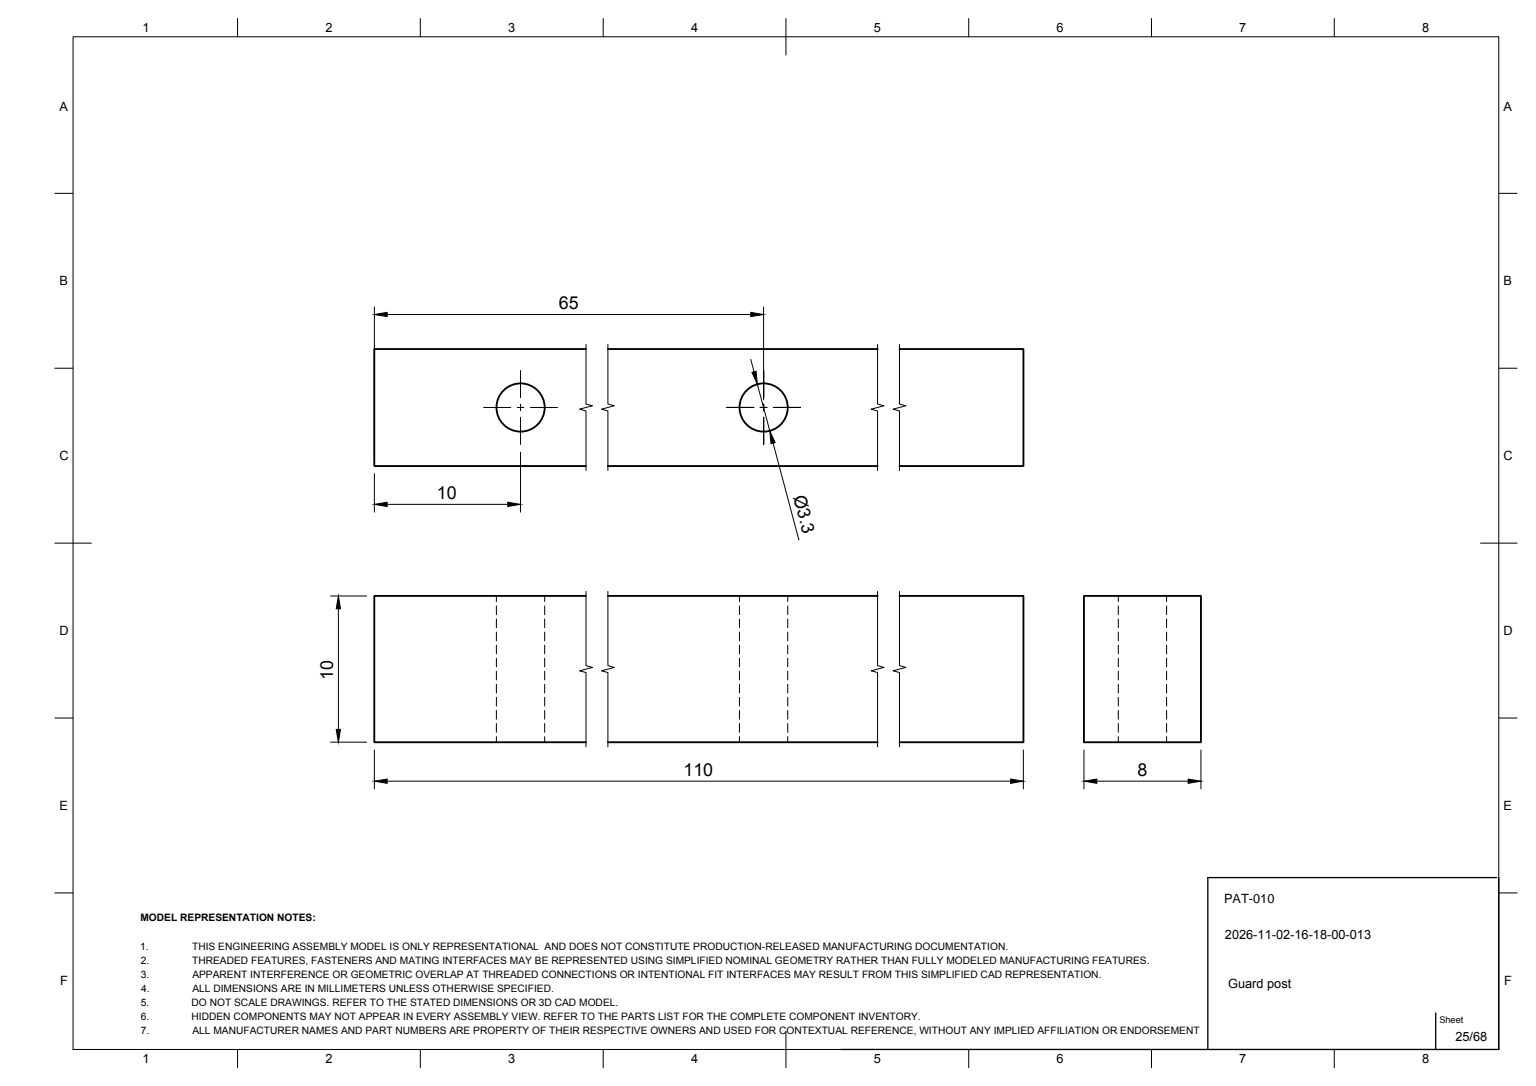
ISO-10303-21;
HEADER;
/* Generated by software containing ST-Developer
 * from STEP Tools, Inc. (www.steptools.com) 
 */

FILE_DESCRIPTION(
/* description */ ('Belt conveyor head drive unit'),
/* implementation_level */ '2;1');

FILE_NAME(
/* name */ 'Guard post.step',
/* time_stamp */ '2026-10-28T03:26:19-07:00',
/* author */ (''),
/* organization */ (''),
/* preprocessor_version */ 'ST-DEVELOPER v20.2',
/* originating_system */ 'Autodesk Translation Framework v15.17.0.0',
/* authorisation */ '');

FILE_SCHEMA (('AUTOMOTIVE_DESIGN { 1 0 10303 214 3 1 1 }'));
ENDSEC;

DATA;
#10=MECHANICAL_DESIGN_GEOMETRIC_PRESENTATION_REPRESENTATION('',(#871),#27069);
#733=SHAPE_REPRESENTATION_RELATIONSHIP('SRR','None',#27377,#802);
#802=ADVANCED_BREP_SHAPE_REPRESENTATION('',(#956),#27019);
#871=STYLED_ITEM('',(#27790),#956);
#956=MANIFOLD_SOLID_BREP('Body1',#13736);
#1135=FACE_BOUND('',#2835,.T.);
#1136=FACE_BOUND('',#2836,.T.);
#1137=FACE_BOUND('',#2839,.T.);
#1138=FACE_BOUND('',#2840,.T.);
#1419=PLANE('',#15151);
#1420=PLANE('',#15152);
#1421=PLANE('',#15153);
#1422=PLANE('',#15154);
#1423=PLANE('',#15155);
#1424=PLANE('',#15156);
#1909=FACE_OUTER_BOUND('',#2832,.T.);
#1910=FACE_OUTER_BOUND('',#2833,.T.);
#1911=FACE_OUTER_BOUND('',#2834,.T.);
#1912=FACE_OUTER_BOUND('',#2837,.T.);
#1913=FACE_OUTER_BOUND('',#2838,.T.);
#1914=FACE_OUTER_BOUND('',#2841,.T.);
#1915=FACE_OUTER_BOUND('',#2842,.T.);
#1916=FACE_OUTER_BOUND('',#2843,.T.);
#2832=EDGE_LOOP('',(#10152,#10153,#10154,#10155));
#2833=EDGE_LOOP('',(#10156,#10157,#10158,#10159));
#2834=EDGE_LOOP('',(#10160,#10161,#10162,#10163));
#2835=EDGE_LOOP('',(#10164));
#2836=EDGE_LOOP('',(#10165));
#2837=EDGE_LOOP('',(#10166,#10167,#10168,#10169));
#2838=EDGE_LOOP('',(#10170,#10171,#10172,#10173));
#2839=EDGE_LOOP('',(#10174));
#2840=EDGE_LOOP('',(#10175));
#2841=EDGE_LOOP('',(#10176,#10177,#10178,#10179));
#2842=EDGE_LOOP('',(#10180,#10181,#10182,#10183));
#2843=EDGE_LOOP('',(#10184,#10185,#10186,#10187));
#3815=LINE('',#22272,#4607);
#3816=LINE('',#22278,#4608);
#3817=LINE('',#22283,#4609);
#3818=LINE('',#22285,#4610);
#3819=LINE('',#22287,#4611);
#3820=LINE('',#22288,#4612);
#3821=LINE('',#22291,#4613);
#3822=LINE('',#22293,#4614);
#3823=LINE('',#22294,#4615);
#3824=LINE('',#22297,#4616);
#3825=LINE('',#22299,#4617);
#3826=LINE('',#22300,#4618);
#3827=LINE('',#22302,#4619);
#3828=LINE('',#22303,#4620);
#4607=VECTOR('',#17921,0.165);
#4608=VECTOR('',#17928,0.165);
#4609=VECTOR('',#17933,1.);
#4610=VECTOR('',#17934,1.);
#4611=VECTOR('',#17935,1.);
#4612=VECTOR('',#17936,1.);
#4613=VECTOR('',#17939,1.);
#4614=VECTOR('',#17940,1.);
#4615=VECTOR('',#17941,1.);
#4616=VECTOR('',#17944,1.);
#4617=VECTOR('',#17945,1.);
#4618=VECTOR('',#17946,1.);
#4619=VECTOR('',#17949,1.);
#4620=VECTOR('',#17950,1.);
#5362=CIRCLE('',#15146,0.165);
#5363=CIRCLE('',#15147,0.165);
#5364=CIRCLE('',#15149,0.165);
#5365=CIRCLE('',#15150,0.165);
#6351=VERTEX_POINT('',#22269);
#6352=VERTEX_POINT('',#22271);
#6353=VERTEX_POINT('',#22275);
#6354=VERTEX_POINT('',#22277);
#6355=VERTEX_POINT('',#22281);
#6356=VERTEX_POINT('',#22282);
#6357=VERTEX_POINT('',#22284);
#6358=VERTEX_POINT('',#22286);
#6359=VERTEX_POINT('',#22290);
#6360=VERTEX_POINT('',#22292);
#6361=VERTEX_POINT('',#22296);
#6362=VERTEX_POINT('',#22298);
#7768=EDGE_CURVE('',#6351,#6351,#5362,.T.);
#7769=EDGE_CURVE('',#6351,#6352,#3815,.T.);
#7770=EDGE_CURVE('',#6352,#6352,#5363,.T.);
#7771=EDGE_CURVE('',#6353,#6353,#5364,.T.);
#7772=EDGE_CURVE('',#6353,#6354,#3816,.T.);
#7773=EDGE_CURVE('',#6354,#6354,#5365,.T.);
#7774=EDGE_CURVE('',#6355,#6356,#3817,.T.);
#7775=EDGE_CURVE('',#6356,#6357,#3818,.T.);
#7776=EDGE_CURVE('',#6358,#6357,#3819,.T.);
#7777=EDGE_CURVE('',#6355,#6358,#3820,.T.);
#7778=EDGE_CURVE('',#6359,#6355,#3821,.T.);
#7779=EDGE_CURVE('',#6360,#6358,#3822,.T.);
#7780=EDGE_CURVE('',#6359,#6360,#3823,.T.);
#7781=EDGE_CURVE('',#6361,#6359,#3824,.T.);
#7782=EDGE_CURVE('',#6362,#6360,#3825,.T.);
#7783=EDGE_CURVE('',#6361,#6362,#3826,.T.);
#7784=EDGE_CURVE('',#6356,#6361,#3827,.T.);
#7785=EDGE_CURVE('',#6357,#6362,#3828,.T.);
#10152=ORIENTED_EDGE('',*,*,#7768,.F.);
#10153=ORIENTED_EDGE('',*,*,#7769,.T.);
#10154=ORIENTED_EDGE('',*,*,#7770,.F.);
#10155=ORIENTED_EDGE('',*,*,#7769,.F.);
#10156=ORIENTED_EDGE('',*,*,#7771,.F.);
#10157=ORIENTED_EDGE('',*,*,#7772,.T.);
#10158=ORIENTED_EDGE('',*,*,#7773,.F.);
#10159=ORIENTED_EDGE('',*,*,#7772,.F.);
#10160=ORIENTED_EDGE('',*,*,#7774,.T.);
#10161=ORIENTED_EDGE('',*,*,#7775,.T.);
#10162=ORIENTED_EDGE('',*,*,#7776,.F.);
#10163=ORIENTED_EDGE('',*,*,#7777,.F.);
#10164=ORIENTED_EDGE('',*,*,#7770,.T.);
#10165=ORIENTED_EDGE('',*,*,#7773,.T.);
#10166=ORIENTED_EDGE('',*,*,#7778,.T.);
#10167=ORIENTED_EDGE('',*,*,#7777,.T.);
#10168=ORIENTED_EDGE('',*,*,#7779,.F.);
#10169=ORIENTED_EDGE('',*,*,#7780,.F.);
#10170=ORIENTED_EDGE('',*,*,#7781,.T.);
#10171=ORIENTED_EDGE('',*,*,#7780,.T.);
#10172=ORIENTED_EDGE('',*,*,#7782,.F.);
#10173=ORIENTED_EDGE('',*,*,#7783,.F.);
#10174=ORIENTED_EDGE('',*,*,#7768,.T.);
#10175=ORIENTED_EDGE('',*,*,#7771,.T.);
#10176=ORIENTED_EDGE('',*,*,#7784,.T.);
#10177=ORIENTED_EDGE('',*,*,#7783,.T.);
#10178=ORIENTED_EDGE('',*,*,#7785,.F.);
#10179=ORIENTED_EDGE('',*,*,#7775,.F.);
#10180=ORIENTED_EDGE('',*,*,#7785,.T.);
#10181=ORIENTED_EDGE('',*,*,#7782,.T.);
#10182=ORIENTED_EDGE('',*,*,#7779,.T.);
#10183=ORIENTED_EDGE('',*,*,#7776,.T.);
#10184=ORIENTED_EDGE('',*,*,#7784,.F.);
#10185=ORIENTED_EDGE('',*,*,#7774,.F.);
#10186=ORIENTED_EDGE('',*,*,#7778,.F.);
#10187=ORIENTED_EDGE('',*,*,#7781,.F.);
#12666=CYLINDRICAL_SURFACE('',#15145,0.165);
#12667=CYLINDRICAL_SURFACE('',#15148,0.165);
#13188=ADVANCED_FACE('',(#1909),#12666,.F.);
#13189=ADVANCED_FACE('',(#1910),#12667,.F.);
#13190=ADVANCED_FACE('',(#1911,#1135,#1136),#1419,.T.);
#13191=ADVANCED_FACE('',(#1912),#1420,.T.);
#13192=ADVANCED_FACE('',(#1913,#1137,#1138),#1421,.T.);
#13193=ADVANCED_FACE('',(#1914),#1422,.T.);
#13194=ADVANCED_FACE('',(#1915),#1423,.T.);
#13195=ADVANCED_FACE('',(#1916),#1424,.F.);
#13736=CLOSED_SHELL('',(#13188,#13189,#13190,#13191,#13192,#13193,#13194,
#13195));
#15144=AXIS2_PLACEMENT_3D('',#22267,#17915,#17916);
#15145=AXIS2_PLACEMENT_3D('',#22268,#17917,#17918);
#15146=AXIS2_PLACEMENT_3D('',#22270,#17919,#17920);
#15147=AXIS2_PLACEMENT_3D('',#22273,#17922,#17923);
#15148=AXIS2_PLACEMENT_3D('',#22274,#17924,#17925);
#15149=AXIS2_PLACEMENT_3D('',#22276,#17926,#17927);
#15150=AXIS2_PLACEMENT_3D('',#22279,#17929,#17930);
#15151=AXIS2_PLACEMENT_3D('',#22280,#17931,#17932);
#15152=AXIS2_PLACEMENT_3D('',#22289,#17937,#17938);
#15153=AXIS2_PLACEMENT_3D('',#22295,#17942,#17943);
#15154=AXIS2_PLACEMENT_3D('',#22301,#17947,#17948);
#15155=AXIS2_PLACEMENT_3D('',#22304,#17951,#17952);
#15156=AXIS2_PLACEMENT_3D('',#22305,#17953,#17954);
#17915=DIRECTION('axis',(0.,0.,1.));
#17916=DIRECTION('refdir',(1.,0.,0.));
#17917=DIRECTION('center_axis',(0.,1.,0.));
#17918=DIRECTION('ref_axis',(1.,0.,0.));
#17919=DIRECTION('center_axis',(0.,1.,0.));
#17920=DIRECTION('ref_axis',(1.,0.,0.));
#17921=DIRECTION('',(0.,1.,0.));
#17922=DIRECTION('center_axis',(0.,-1.,0.));
#17923=DIRECTION('ref_axis',(1.,0.,0.));
#17924=DIRECTION('center_axis',(0.,1.,0.));
#17925=DIRECTION('ref_axis',(1.,0.,0.));
#17926=DIRECTION('center_axis',(0.,1.,0.));
#17927=DIRECTION('ref_axis',(1.,0.,0.));
#17928=DIRECTION('',(0.,1.,0.));
#17929=DIRECTION('center_axis',(0.,-1.,0.));
#17930=DIRECTION('ref_axis',(1.,0.,0.));
#17931=DIRECTION('center_axis',(0.,1.,0.));
#17932=DIRECTION('ref_axis',(-1.,0.,0.));
#17933=DIRECTION('',(-1.,0.,0.));
#17934=DIRECTION('',(0.,0.,1.));
#17935=DIRECTION('',(-1.,0.,0.));
#17936=DIRECTION('',(0.,0.,1.));
#17937=DIRECTION('center_axis',(1.,0.,0.));
#17938=DIRECTION('ref_axis',(0.,1.,0.));
#17939=DIRECTION('',(0.,1.,0.));
#17940=DIRECTION('',(0.,1.,0.));
#17941=DIRECTION('',(0.,0.,1.));
#17942=DIRECTION('center_axis',(0.,-1.,0.));
#17943=DIRECTION('ref_axis',(1.,0.,0.));
#17944=DIRECTION('',(1.,0.,0.));
#17945=DIRECTION('',(1.,0.,0.));
#17946=DIRECTION('',(0.,0.,1.));
#17947=DIRECTION('center_axis',(-1.,0.,0.));
#17948=DIRECTION('ref_axis',(0.,-1.,0.));
#17949=DIRECTION('',(0.,-1.,0.));
#17950=DIRECTION('',(0.,-1.,0.));
#17951=DIRECTION('center_axis',(0.,0.,1.));
#17952=DIRECTION('ref_axis',(1.,0.,0.));
#17953=DIRECTION('center_axis',(0.,0.,1.));
#17954=DIRECTION('ref_axis',(1.,0.,0.));
#22267=CARTESIAN_POINT('',(0.,0.,0.));
#22268=CARTESIAN_POINT('Origin',(-3.,-6.1,4.5));
#22269=CARTESIAN_POINT('',(-3.165,-6.,4.5));
#22270=CARTESIAN_POINT('Origin',(-3.,-6.,4.5));
#22271=CARTESIAN_POINT('',(-3.165,-5.,4.5));
#22272=CARTESIAN_POINT('',(-3.165,-6.1,4.5));
#22273=CARTESIAN_POINT('Origin',(-3.,-5.,4.5));
#22274=CARTESIAN_POINT('Origin',(-3.,-6.1,10.));
#22275=CARTESIAN_POINT('',(-3.165,-6.,10.));
#22276=CARTESIAN_POINT('Origin',(-3.,-6.,10.));
#22277=CARTESIAN_POINT('',(-3.165,-5.,10.));
#22278=CARTESIAN_POINT('',(-3.165,-6.1,10.));
#22279=CARTESIAN_POINT('Origin',(-3.,-5.,10.));
#22280=CARTESIAN_POINT('Origin',(-2.6,-5.,0.));
#22281=CARTESIAN_POINT('',(-2.6,-5.,0.));
#22282=CARTESIAN_POINT('',(-3.4,-5.,0.));
#22283=CARTESIAN_POINT('',(-2.6,-5.,0.));
#22284=CARTESIAN_POINT('',(-3.4,-5.,11.));
#22285=CARTESIAN_POINT('',(-3.4,-5.,0.));
#22286=CARTESIAN_POINT('',(-2.6,-5.,11.));
#22287=CARTESIAN_POINT('',(-2.6,-5.,11.));
#22288=CARTESIAN_POINT('',(-2.6,-5.,0.));
#22289=CARTESIAN_POINT('Origin',(-2.6,-6.,0.));
#22290=CARTESIAN_POINT('',(-2.6,-6.,0.));
#22291=CARTESIAN_POINT('',(-2.6,-6.,0.));
#22292=CARTESIAN_POINT('',(-2.6,-6.,11.));
#22293=CARTESIAN_POINT('',(-2.6,-6.,11.));
#22294=CARTESIAN_POINT('',(-2.6,-6.,0.));
#22295=CARTESIAN_POINT('Origin',(-3.4,-6.,0.));
#22296=CARTESIAN_POINT('',(-3.4,-6.,0.));
#22297=CARTESIAN_POINT('',(-3.4,-6.,0.));
#22298=CARTESIAN_POINT('',(-3.4,-6.,11.));
#22299=CARTESIAN_POINT('',(-3.4,-6.,11.));
#22300=CARTESIAN_POINT('',(-3.4,-6.,0.));
#22301=CARTESIAN_POINT('Origin',(-3.4,-5.,0.));
#22302=CARTESIAN_POINT('',(-3.4,-5.,0.));
#22303=CARTESIAN_POINT('',(-3.4,-5.,11.));
#22304=CARTESIAN_POINT('Origin',(-3.,-5.5,11.));
#22305=CARTESIAN_POINT('Origin',(-3.,-5.5,0.));
#26942=UNCERTAINTY_MEASURE_WITH_UNIT(LENGTH_MEASURE(0.001),#27070,
'DISTANCE_ACCURACY_VALUE',
'Maximum model space distance between geometric entities at asserted c
onnectivities');
#26992=UNCERTAINTY_MEASURE_WITH_UNIT(LENGTH_MEASURE(0.001),#27070,
'DISTANCE_ACCURACY_VALUE',
'Maximum model space distance between geometric entities at asserted c
onnectivities');
#27019=(
GEOMETRIC_REPRESENTATION_CONTEXT(3)
GLOBAL_UNCERTAINTY_ASSIGNED_CONTEXT((#26942))
GLOBAL_UNIT_ASSIGNED_CONTEXT((#27070,#27072,#27073))
REPRESENTATION_CONTEXT('','3D')
);
#27069=(
GEOMETRIC_REPRESENTATION_CONTEXT(3)
GLOBAL_UNCERTAINTY_ASSIGNED_CONTEXT((#26992))
GLOBAL_UNIT_ASSIGNED_CONTEXT((#27070,#27072,#27073))
REPRESENTATION_CONTEXT('','3D')
);
#27070=(
LENGTH_UNIT()
NAMED_UNIT(*)
SI_UNIT(.CENTI.,.METRE.)
);
#27072=(
NAMED_UNIT(*)
PLANE_ANGLE_UNIT()
SI_UNIT($,.RADIAN.)
);
#27073=(
NAMED_UNIT(*)
SI_UNIT($,.STERADIAN.)
SOLID_ANGLE_UNIT()
);
#27100=SHAPE_DEFINITION_REPRESENTATION(#27176,#27377);
#27176=PRODUCT_DEFINITION_SHAPE('',$,#27454);
#27377=SHAPE_REPRESENTATION('',(#15144),#27019);
#27427=PRODUCT_DEFINITION_CONTEXT('part definition',#27657,'design');
#27454=PRODUCT_DEFINITION('Guard post','Guard post',#27530,#27427);
#27530=PRODUCT_DEFINITION_FORMATION('',$,#27685);
#27657=APPLICATION_CONTEXT(
'Core Data for Automotive Mechanical Design Process');
#27658=PRODUCT_CONTEXT('part definition',#27657,'mechanical');
#27685=PRODUCT('Guard post','Guard post','Guard post',(#27658));
#27784=COLOUR_RGB('Sky Blue',0.24,0.69,0.87);
#27785=FILL_AREA_STYLE_COLOUR('',#27784);
#27786=FILL_AREA_STYLE('',(#27785));
#27787=SURFACE_STYLE_FILL_AREA(#27786);
#27788=SURFACE_SIDE_STYLE('',(#27787));
#27789=SURFACE_STYLE_USAGE(.BOTH.,#27788);
#27790=PRESENTATION_STYLE_ASSIGNMENT((#27789));
ENDSEC;
END-ISO-10303-21;
